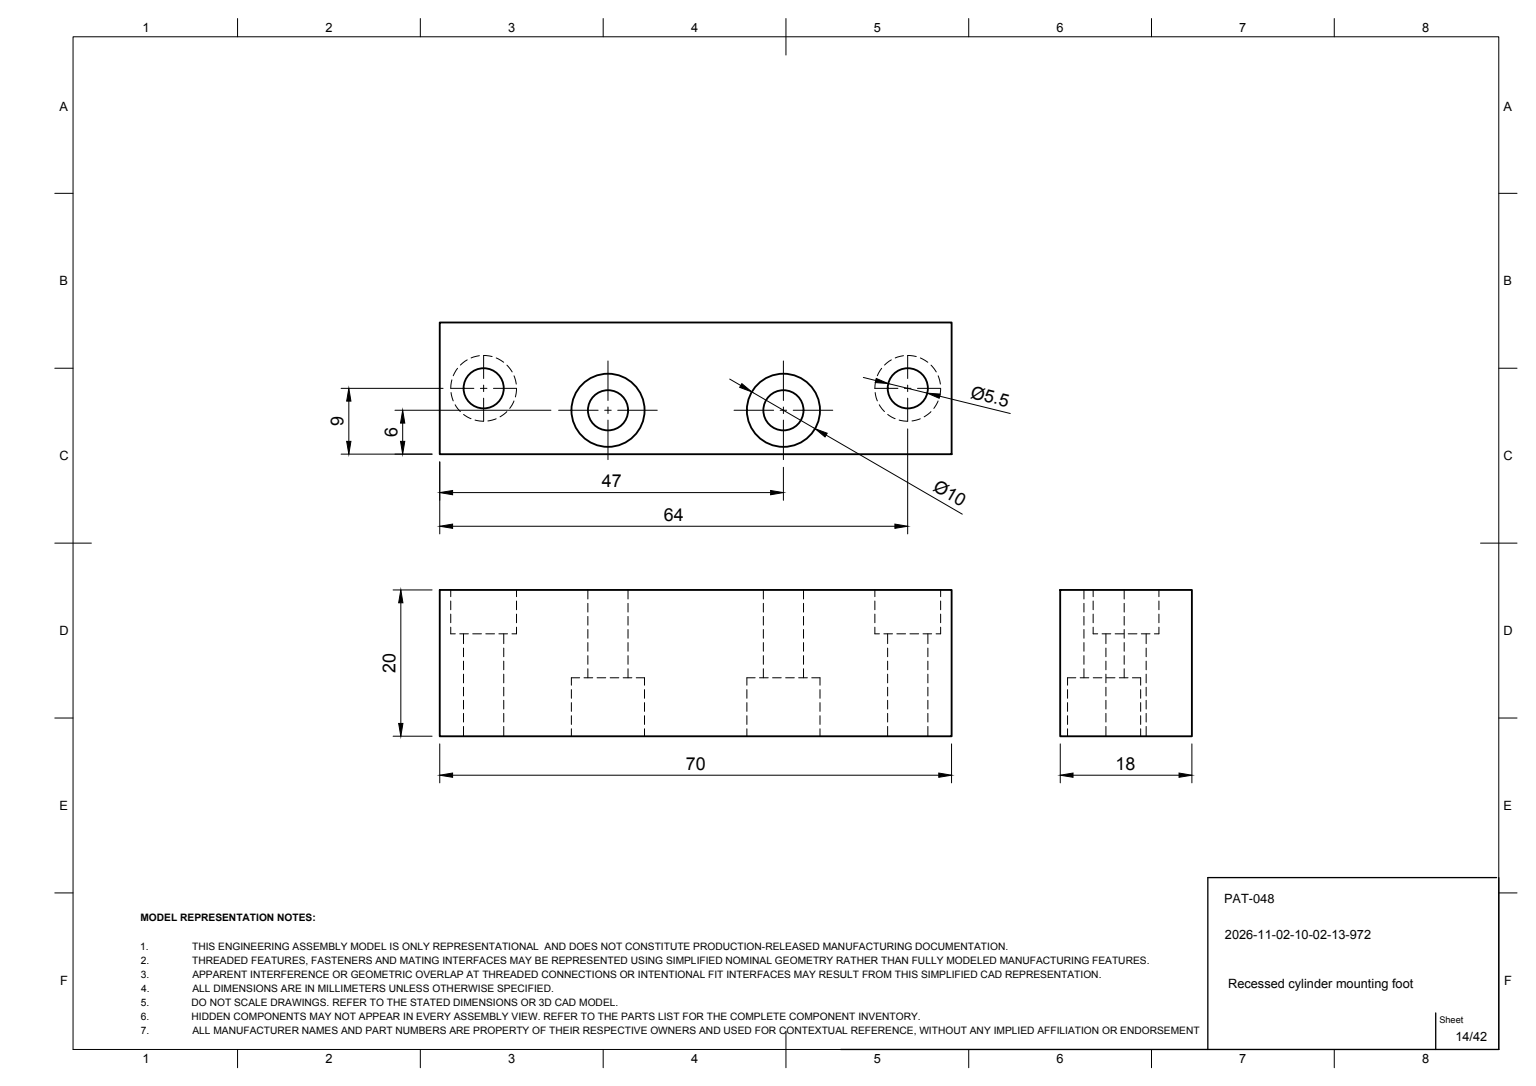
ISO-10303-21;
HEADER;
/* Generated by software containing ST-Developer
 * from STEP Tools, Inc. (www.steptools.com) 
 */

FILE_DESCRIPTION(
/* description */ ('Guided pneumatic stop gate'),
/* implementation_level */ '2;1');

FILE_NAME(
/* name */ 'Recessed cylinder mounting foot.step',
/* time_stamp */ '2026-10-27T21:43:45-07:00',
/* author */ (''),
/* organization */ (''),
/* preprocessor_version */ 'ST-DEVELOPER v20.2',
/* originating_system */ 'Autodesk Translation Framework v15.17.0.0',
/* authorisation */ '');

FILE_SCHEMA (('AUTOMOTIVE_DESIGN { 1 0 10303 214 3 1 1 }'));
ENDSEC;

DATA;
#10=MECHANICAL_DESIGN_GEOMETRIC_PRESENTATION_REPRESENTATION('',(#544),#14392);
#460=SHAPE_REPRESENTATION_RELATIONSHIP('SRR','None',#14594,#502);
#502=ADVANCED_BREP_SHAPE_REPRESENTATION('',(#586),#14356);
#544=STYLED_ITEM('',(#14877),#586);
#586=MANIFOLD_SOLID_BREP('Body1',#7884);
#669=FACE_BOUND('',#1794,.T.);
#670=FACE_BOUND('',#1797,.T.);
#671=FACE_BOUND('',#1802,.T.);
#672=FACE_BOUND('',#1805,.T.);
#673=FACE_BOUND('',#1813,.T.);
#674=FACE_BOUND('',#1814,.T.);
#675=FACE_BOUND('',#1815,.T.);
#676=FACE_BOUND('',#1816,.T.);
#677=FACE_BOUND('',#1818,.T.);
#678=FACE_BOUND('',#1819,.T.);
#679=FACE_BOUND('',#1820,.T.);
#680=FACE_BOUND('',#1821,.T.);
#927=PLANE('',#8666);
#928=PLANE('',#8671);
#929=PLANE('',#8680);
#930=PLANE('',#8685);
#931=PLANE('',#8691);
#932=PLANE('',#8692);
#933=PLANE('',#8693);
#934=PLANE('',#8694);
#935=PLANE('',#8695);
#936=PLANE('',#8696);
#1263=FACE_OUTER_BOUND('',#1792,.T.);
#1264=FACE_OUTER_BOUND('',#1793,.T.);
#1265=FACE_OUTER_BOUND('',#1795,.T.);
#1266=FACE_OUTER_BOUND('',#1796,.T.);
#1267=FACE_OUTER_BOUND('',#1798,.T.);
#1268=FACE_OUTER_BOUND('',#1799,.T.);
#1269=FACE_OUTER_BOUND('',#1800,.T.);
#1270=FACE_OUTER_BOUND('',#1801,.T.);
#1271=FACE_OUTER_BOUND('',#1803,.T.);
#1272=FACE_OUTER_BOUND('',#1804,.T.);
#1273=FACE_OUTER_BOUND('',#1806,.T.);
#1274=FACE_OUTER_BOUND('',#1807,.T.);
#1275=FACE_OUTER_BOUND('',#1808,.T.);
#1276=FACE_OUTER_BOUND('',#1809,.T.);
#1277=FACE_OUTER_BOUND('',#1810,.T.);
#1278=FACE_OUTER_BOUND('',#1811,.T.);
#1279=FACE_OUTER_BOUND('',#1812,.T.);
#1280=FACE_OUTER_BOUND('',#1817,.T.);
#1792=EDGE_LOOP('',(#5898,#5899,#5900,#5901));
#1793=EDGE_LOOP('',(#5902));
#1794=EDGE_LOOP('',(#5903));
#1795=EDGE_LOOP('',(#5904,#5905,#5906,#5907));
#1796=EDGE_LOOP('',(#5908));
#1797=EDGE_LOOP('',(#5909));
#1798=EDGE_LOOP('',(#5910,#5911,#5912,#5913));
#1799=EDGE_LOOP('',(#5914,#5915,#5916,#5917));
#1800=EDGE_LOOP('',(#5918,#5919,#5920,#5921));
#1801=EDGE_LOOP('',(#5922));
#1802=EDGE_LOOP('',(#5923));
#1803=EDGE_LOOP('',(#5924,#5925,#5926,#5927));
#1804=EDGE_LOOP('',(#5928));
#1805=EDGE_LOOP('',(#5929));
#1806=EDGE_LOOP('',(#5930,#5931,#5932,#5933));
#1807=EDGE_LOOP('',(#5934,#5935,#5936,#5937));
#1808=EDGE_LOOP('',(#5938,#5939,#5940,#5941));
#1809=EDGE_LOOP('',(#5942,#5943,#5944,#5945));
#1810=EDGE_LOOP('',(#5946,#5947,#5948,#5949));
#1811=EDGE_LOOP('',(#5950,#5951,#5952,#5953));
#1812=EDGE_LOOP('',(#5954,#5955,#5956,#5957));
#1813=EDGE_LOOP('',(#5958));
#1814=EDGE_LOOP('',(#5959));
#1815=EDGE_LOOP('',(#5960));
#1816=EDGE_LOOP('',(#5961));
#1817=EDGE_LOOP('',(#5962,#5963,#5964,#5965));
#1818=EDGE_LOOP('',(#5966));
#1819=EDGE_LOOP('',(#5967));
#1820=EDGE_LOOP('',(#5968));
#1821=EDGE_LOOP('',(#5969));
#2447=LINE('',#12554,#2992);
#2448=LINE('',#12563,#2993);
#2449=LINE('',#12571,#2994);
#2450=LINE('',#12575,#2995);
#2451=LINE('',#12580,#2996);
#2452=LINE('',#12589,#2997);
#2453=LINE('',#12596,#2998);
#2454=LINE('',#12600,#2999);
#2455=LINE('',#12605,#3000);
#2456=LINE('',#12607,#3001);
#2457=LINE('',#12609,#3002);
#2458=LINE('',#12610,#3003);
#2459=LINE('',#12613,#3004);
#2460=LINE('',#12615,#3005);
#2461=LINE('',#12616,#3006);
#2462=LINE('',#12619,#3007);
#2463=LINE('',#12621,#3008);
#2464=LINE('',#12622,#3009);
#2465=LINE('',#12624,#3010);
#2466=LINE('',#12625,#3011);
#2992=VECTOR('',#10112,0.45);
#2993=VECTOR('',#10123,0.45);
#2994=VECTOR('',#10134,0.275);
#2995=VECTOR('',#10139,0.275);
#2996=VECTOR('',#10144,0.5);
#2997=VECTOR('',#10155,0.5);
#2998=VECTOR('',#10164,0.275);
#2999=VECTOR('',#10169,0.275);
#3000=VECTOR('',#10174,1.);
#3001=VECTOR('',#10175,1.);
#3002=VECTOR('',#10176,1.);
#3003=VECTOR('',#10177,1.);
#3004=VECTOR('',#10180,1.);
#3005=VECTOR('',#10181,1.);
#3006=VECTOR('',#10182,1.);
#3007=VECTOR('',#10185,1.);
#3008=VECTOR('',#10186,1.);
#3009=VECTOR('',#10187,1.);
#3010=VECTOR('',#10190,1.);
#3011=VECTOR('',#10191,1.);
#3476=CIRCLE('',#8664,0.45);
#3477=CIRCLE('',#8665,0.45);
#3478=CIRCLE('',#8667,0.275);
#3479=CIRCLE('',#8669,0.45);
#3480=CIRCLE('',#8670,0.45);
#3481=CIRCLE('',#8672,0.275);
#3482=CIRCLE('',#8674,0.275);
#3483=CIRCLE('',#8676,0.275);
#3484=CIRCLE('',#8678,0.5);
#3485=CIRCLE('',#8679,0.5);
#3486=CIRCLE('',#8681,0.275);
#3487=CIRCLE('',#8683,0.5);
#3488=CIRCLE('',#8684,0.5);
#3489=CIRCLE('',#8686,0.275);
#3490=CIRCLE('',#8688,0.275);
#3491=CIRCLE('',#8690,0.275);
#3919=VERTEX_POINT('',#12551);
#3920=VERTEX_POINT('',#12553);
#3921=VERTEX_POINT('',#12557);
#3922=VERTEX_POINT('',#12560);
#3923=VERTEX_POINT('',#12562);
#3924=VERTEX_POINT('',#12566);
#3925=VERTEX_POINT('',#12569);
#3926=VERTEX_POINT('',#12573);
#3927=VERTEX_POINT('',#12577);
#3928=VERTEX_POINT('',#12579);
#3929=VERTEX_POINT('',#12583);
#3930=VERTEX_POINT('',#12586);
#3931=VERTEX_POINT('',#12588);
#3932=VERTEX_POINT('',#12592);
#3933=VERTEX_POINT('',#12595);
#3934=VERTEX_POINT('',#12599);
#3935=VERTEX_POINT('',#12603);
#3936=VERTEX_POINT('',#12604);
#3937=VERTEX_POINT('',#12606);
#3938=VERTEX_POINT('',#12608);
#3939=VERTEX_POINT('',#12612);
#3940=VERTEX_POINT('',#12614);
#3941=VERTEX_POINT('',#12618);
#3942=VERTEX_POINT('',#12620);
#4647=EDGE_CURVE('',#3919,#3919,#3476,.T.);
#4648=EDGE_CURVE('',#3919,#3920,#2447,.T.);
#4649=EDGE_CURVE('',#3920,#3920,#3477,.T.);
#4650=EDGE_CURVE('',#3921,#3921,#3478,.T.);
#4651=EDGE_CURVE('',#3922,#3922,#3479,.T.);
#4652=EDGE_CURVE('',#3922,#3923,#2448,.T.);
#4653=EDGE_CURVE('',#3923,#3923,#3480,.T.);
#4654=EDGE_CURVE('',#3924,#3924,#3481,.T.);
#4655=EDGE_CURVE('',#3925,#3925,#3482,.T.);
#4656=EDGE_CURVE('',#3925,#3921,#2449,.T.);
#4657=EDGE_CURVE('',#3926,#3926,#3483,.T.);
#4658=EDGE_CURVE('',#3926,#3924,#2450,.T.);
#4659=EDGE_CURVE('',#3927,#3927,#3484,.T.);
#4660=EDGE_CURVE('',#3927,#3928,#2451,.T.);
#4661=EDGE_CURVE('',#3928,#3928,#3485,.T.);
#4662=EDGE_CURVE('',#3929,#3929,#3486,.T.);
#4663=EDGE_CURVE('',#3930,#3930,#3487,.T.);
#4664=EDGE_CURVE('',#3930,#3931,#2452,.T.);
#4665=EDGE_CURVE('',#3931,#3931,#3488,.T.);
#4666=EDGE_CURVE('',#3932,#3932,#3489,.T.);
#4667=EDGE_CURVE('',#3929,#3933,#2453,.T.);
#4668=EDGE_CURVE('',#3933,#3933,#3490,.T.);
#4669=EDGE_CURVE('',#3932,#3934,#2454,.T.);
#4670=EDGE_CURVE('',#3934,#3934,#3491,.T.);
#4671=EDGE_CURVE('',#3935,#3936,#2455,.T.);
#4672=EDGE_CURVE('',#3936,#3937,#2456,.T.);
#4673=EDGE_CURVE('',#3938,#3937,#2457,.T.);
#4674=EDGE_CURVE('',#3935,#3938,#2458,.T.);
#4675=EDGE_CURVE('',#3939,#3935,#2459,.T.);
#4676=EDGE_CURVE('',#3940,#3938,#2460,.T.);
#4677=EDGE_CURVE('',#3939,#3940,#2461,.T.);
#4678=EDGE_CURVE('',#3941,#3939,#2462,.T.);
#4679=EDGE_CURVE('',#3942,#3940,#2463,.T.);
#4680=EDGE_CURVE('',#3941,#3942,#2464,.T.);
#4681=EDGE_CURVE('',#3936,#3941,#2465,.T.);
#4682=EDGE_CURVE('',#3937,#3942,#2466,.T.);
#5898=ORIENTED_EDGE('',*,*,#4647,.F.);
#5899=ORIENTED_EDGE('',*,*,#4648,.T.);
#5900=ORIENTED_EDGE('',*,*,#4649,.F.);
#5901=ORIENTED_EDGE('',*,*,#4648,.F.);
#5902=ORIENTED_EDGE('',*,*,#4647,.T.);
#5903=ORIENTED_EDGE('',*,*,#4650,.F.);
#5904=ORIENTED_EDGE('',*,*,#4651,.F.);
#5905=ORIENTED_EDGE('',*,*,#4652,.T.);
#5906=ORIENTED_EDGE('',*,*,#4653,.F.);
#5907=ORIENTED_EDGE('',*,*,#4652,.F.);
#5908=ORIENTED_EDGE('',*,*,#4651,.T.);
#5909=ORIENTED_EDGE('',*,*,#4654,.F.);
#5910=ORIENTED_EDGE('',*,*,#4655,.F.);
#5911=ORIENTED_EDGE('',*,*,#4656,.T.);
#5912=ORIENTED_EDGE('',*,*,#4650,.T.);
#5913=ORIENTED_EDGE('',*,*,#4656,.F.);
#5914=ORIENTED_EDGE('',*,*,#4657,.F.);
#5915=ORIENTED_EDGE('',*,*,#4658,.T.);
#5916=ORIENTED_EDGE('',*,*,#4654,.T.);
#5917=ORIENTED_EDGE('',*,*,#4658,.F.);
#5918=ORIENTED_EDGE('',*,*,#4659,.F.);
#5919=ORIENTED_EDGE('',*,*,#4660,.T.);
#5920=ORIENTED_EDGE('',*,*,#4661,.T.);
#5921=ORIENTED_EDGE('',*,*,#4660,.F.);
#5922=ORIENTED_EDGE('',*,*,#4661,.F.);
#5923=ORIENTED_EDGE('',*,*,#4662,.F.);
#5924=ORIENTED_EDGE('',*,*,#4663,.F.);
#5925=ORIENTED_EDGE('',*,*,#4664,.T.);
#5926=ORIENTED_EDGE('',*,*,#4665,.T.);
#5927=ORIENTED_EDGE('',*,*,#4664,.F.);
#5928=ORIENTED_EDGE('',*,*,#4665,.F.);
#5929=ORIENTED_EDGE('',*,*,#4666,.F.);
#5930=ORIENTED_EDGE('',*,*,#4662,.T.);
#5931=ORIENTED_EDGE('',*,*,#4667,.T.);
#5932=ORIENTED_EDGE('',*,*,#4668,.F.);
#5933=ORIENTED_EDGE('',*,*,#4667,.F.);
#5934=ORIENTED_EDGE('',*,*,#4666,.T.);
#5935=ORIENTED_EDGE('',*,*,#4669,.T.);
#5936=ORIENTED_EDGE('',*,*,#4670,.F.);
#5937=ORIENTED_EDGE('',*,*,#4669,.F.);
#5938=ORIENTED_EDGE('',*,*,#4671,.T.);
#5939=ORIENTED_EDGE('',*,*,#4672,.T.);
#5940=ORIENTED_EDGE('',*,*,#4673,.F.);
#5941=ORIENTED_EDGE('',*,*,#4674,.F.);
#5942=ORIENTED_EDGE('',*,*,#4675,.T.);
#5943=ORIENTED_EDGE('',*,*,#4674,.T.);
#5944=ORIENTED_EDGE('',*,*,#4676,.F.);
#5945=ORIENTED_EDGE('',*,*,#4677,.F.);
#5946=ORIENTED_EDGE('',*,*,#4678,.T.);
#5947=ORIENTED_EDGE('',*,*,#4677,.T.);
#5948=ORIENTED_EDGE('',*,*,#4679,.F.);
#5949=ORIENTED_EDGE('',*,*,#4680,.F.);
#5950=ORIENTED_EDGE('',*,*,#4681,.T.);
#5951=ORIENTED_EDGE('',*,*,#4680,.T.);
#5952=ORIENTED_EDGE('',*,*,#4682,.F.);
#5953=ORIENTED_EDGE('',*,*,#4672,.F.);
#5954=ORIENTED_EDGE('',*,*,#4682,.T.);
#5955=ORIENTED_EDGE('',*,*,#4679,.T.);
#5956=ORIENTED_EDGE('',*,*,#4676,.T.);
#5957=ORIENTED_EDGE('',*,*,#4673,.T.);
#5958=ORIENTED_EDGE('',*,*,#4649,.T.);
#5959=ORIENTED_EDGE('',*,*,#4653,.T.);
#5960=ORIENTED_EDGE('',*,*,#4668,.T.);
#5961=ORIENTED_EDGE('',*,*,#4670,.T.);
#5962=ORIENTED_EDGE('',*,*,#4681,.F.);
#5963=ORIENTED_EDGE('',*,*,#4671,.F.);
#5964=ORIENTED_EDGE('',*,*,#4675,.F.);
#5965=ORIENTED_EDGE('',*,*,#4678,.F.);
#5966=ORIENTED_EDGE('',*,*,#4655,.T.);
#5967=ORIENTED_EDGE('',*,*,#4657,.T.);
#5968=ORIENTED_EDGE('',*,*,#4659,.T.);
#5969=ORIENTED_EDGE('',*,*,#4663,.T.);
#7289=CYLINDRICAL_SURFACE('',#8663,0.45);
#7290=CYLINDRICAL_SURFACE('',#8668,0.45);
#7291=CYLINDRICAL_SURFACE('',#8673,0.275);
#7292=CYLINDRICAL_SURFACE('',#8675,0.275);
#7293=CYLINDRICAL_SURFACE('',#8677,0.5);
#7294=CYLINDRICAL_SURFACE('',#8682,0.5);
#7295=CYLINDRICAL_SURFACE('',#8687,0.275);
#7296=CYLINDRICAL_SURFACE('',#8689,0.275);
#7545=ADVANCED_FACE('',(#1263),#7289,.F.);
#7546=ADVANCED_FACE('',(#1264,#669),#927,.T.);
#7547=ADVANCED_FACE('',(#1265),#7290,.F.);
#7548=ADVANCED_FACE('',(#1266,#670),#928,.T.);
#7549=ADVANCED_FACE('',(#1267),#7291,.F.);
#7550=ADVANCED_FACE('',(#1268),#7292,.F.);
#7551=ADVANCED_FACE('',(#1269),#7293,.F.);
#7552=ADVANCED_FACE('',(#1270,#671),#929,.F.);
#7553=ADVANCED_FACE('',(#1271),#7294,.F.);
#7554=ADVANCED_FACE('',(#1272,#672),#930,.F.);
#7555=ADVANCED_FACE('',(#1273),#7295,.F.);
#7556=ADVANCED_FACE('',(#1274),#7296,.F.);
#7557=ADVANCED_FACE('',(#1275),#931,.T.);
#7558=ADVANCED_FACE('',(#1276),#932,.T.);
#7559=ADVANCED_FACE('',(#1277),#933,.T.);
#7560=ADVANCED_FACE('',(#1278),#934,.T.);
#7561=ADVANCED_FACE('',(#1279,#673,#674,#675,#676),#935,.T.);
#7562=ADVANCED_FACE('',(#1280,#677,#678,#679,#680),#936,.F.);
#7884=CLOSED_SHELL('',(#7545,#7546,#7547,#7548,#7549,#7550,#7551,#7552,
#7553,#7554,#7555,#7556,#7557,#7558,#7559,#7560,#7561,#7562));
#8662=AXIS2_PLACEMENT_3D('',#12549,#10106,#10107);
#8663=AXIS2_PLACEMENT_3D('',#12550,#10108,#10109);
#8664=AXIS2_PLACEMENT_3D('',#12552,#10110,#10111);
#8665=AXIS2_PLACEMENT_3D('',#12555,#10113,#10114);
#8666=AXIS2_PLACEMENT_3D('',#12556,#10115,#10116);
#8667=AXIS2_PLACEMENT_3D('',#12558,#10117,#10118);
#8668=AXIS2_PLACEMENT_3D('',#12559,#10119,#10120);
#8669=AXIS2_PLACEMENT_3D('',#12561,#10121,#10122);
#8670=AXIS2_PLACEMENT_3D('',#12564,#10124,#10125);
#8671=AXIS2_PLACEMENT_3D('',#12565,#10126,#10127);
#8672=AXIS2_PLACEMENT_3D('',#12567,#10128,#10129);
#8673=AXIS2_PLACEMENT_3D('',#12568,#10130,#10131);
#8674=AXIS2_PLACEMENT_3D('',#12570,#10132,#10133);
#8675=AXIS2_PLACEMENT_3D('',#12572,#10135,#10136);
#8676=AXIS2_PLACEMENT_3D('',#12574,#10137,#10138);
#8677=AXIS2_PLACEMENT_3D('',#12576,#10140,#10141);
#8678=AXIS2_PLACEMENT_3D('',#12578,#10142,#10143);
#8679=AXIS2_PLACEMENT_3D('',#12581,#10145,#10146);
#8680=AXIS2_PLACEMENT_3D('',#12582,#10147,#10148);
#8681=AXIS2_PLACEMENT_3D('',#12584,#10149,#10150);
#8682=AXIS2_PLACEMENT_3D('',#12585,#10151,#10152);
#8683=AXIS2_PLACEMENT_3D('',#12587,#10153,#10154);
#8684=AXIS2_PLACEMENT_3D('',#12590,#10156,#10157);
#8685=AXIS2_PLACEMENT_3D('',#12591,#10158,#10159);
#8686=AXIS2_PLACEMENT_3D('',#12593,#10160,#10161);
#8687=AXIS2_PLACEMENT_3D('',#12594,#10162,#10163);
#8688=AXIS2_PLACEMENT_3D('',#12597,#10165,#10166);
#8689=AXIS2_PLACEMENT_3D('',#12598,#10167,#10168);
#8690=AXIS2_PLACEMENT_3D('',#12601,#10170,#10171);
#8691=AXIS2_PLACEMENT_3D('',#12602,#10172,#10173);
#8692=AXIS2_PLACEMENT_3D('',#12611,#10178,#10179);
#8693=AXIS2_PLACEMENT_3D('',#12617,#10183,#10184);
#8694=AXIS2_PLACEMENT_3D('',#12623,#10188,#10189);
#8695=AXIS2_PLACEMENT_3D('',#12626,#10192,#10193);
#8696=AXIS2_PLACEMENT_3D('',#12627,#10194,#10195);
#10106=DIRECTION('axis',(0.,0.,1.));
#10107=DIRECTION('refdir',(1.,0.,0.));
#10108=DIRECTION('center_axis',(0.,0.,1.));
#10109=DIRECTION('ref_axis',(1.,0.,0.));
#10110=DIRECTION('center_axis',(0.,0.,1.));
#10111=DIRECTION('ref_axis',(1.,0.,0.));
#10112=DIRECTION('',(0.,0.,1.));
#10113=DIRECTION('center_axis',(0.,0.,-1.));
#10114=DIRECTION('ref_axis',(1.,0.,0.));
#10115=DIRECTION('center_axis',(0.,0.,1.));
#10116=DIRECTION('ref_axis',(1.,0.,0.));
#10117=DIRECTION('center_axis',(0.,0.,1.));
#10118=DIRECTION('ref_axis',(1.,0.,0.));
#10119=DIRECTION('center_axis',(0.,0.,1.));
#10120=DIRECTION('ref_axis',(1.,0.,0.));
#10121=DIRECTION('center_axis',(0.,0.,1.));
#10122=DIRECTION('ref_axis',(1.,0.,0.));
#10123=DIRECTION('',(0.,0.,1.));
#10124=DIRECTION('center_axis',(0.,0.,-1.));
#10125=DIRECTION('ref_axis',(1.,0.,0.));
#10126=DIRECTION('center_axis',(0.,0.,1.));
#10127=DIRECTION('ref_axis',(1.,0.,0.));
#10128=DIRECTION('center_axis',(0.,0.,1.));
#10129=DIRECTION('ref_axis',(1.,0.,0.));
#10130=DIRECTION('center_axis',(0.,0.,1.));
#10131=DIRECTION('ref_axis',(1.,0.,0.));
#10132=DIRECTION('center_axis',(0.,0.,1.));
#10133=DIRECTION('ref_axis',(1.,0.,0.));
#10134=DIRECTION('',(0.,0.,1.));
#10135=DIRECTION('center_axis',(0.,0.,1.));
#10136=DIRECTION('ref_axis',(1.,0.,0.));
#10137=DIRECTION('center_axis',(0.,0.,1.));
#10138=DIRECTION('ref_axis',(1.,0.,0.));
#10139=DIRECTION('',(0.,0.,1.));
#10140=DIRECTION('center_axis',(0.,0.,1.));
#10141=DIRECTION('ref_axis',(1.,0.,0.));
#10142=DIRECTION('center_axis',(0.,0.,1.));
#10143=DIRECTION('ref_axis',(1.,0.,0.));
#10144=DIRECTION('',(0.,0.,1.));
#10145=DIRECTION('center_axis',(0.,0.,1.));
#10146=DIRECTION('ref_axis',(1.,0.,0.));
#10147=DIRECTION('center_axis',(0.,0.,1.));
#10148=DIRECTION('ref_axis',(1.,0.,0.));
#10149=DIRECTION('center_axis',(0.,0.,-1.));
#10150=DIRECTION('ref_axis',(1.,0.,0.));
#10151=DIRECTION('center_axis',(0.,0.,1.));
#10152=DIRECTION('ref_axis',(1.,0.,0.));
#10153=DIRECTION('center_axis',(0.,0.,1.));
#10154=DIRECTION('ref_axis',(1.,0.,0.));
#10155=DIRECTION('',(0.,0.,1.));
#10156=DIRECTION('center_axis',(0.,0.,1.));
#10157=DIRECTION('ref_axis',(1.,0.,0.));
#10158=DIRECTION('center_axis',(0.,0.,1.));
#10159=DIRECTION('ref_axis',(1.,0.,0.));
#10160=DIRECTION('center_axis',(0.,0.,-1.));
#10161=DIRECTION('ref_axis',(1.,0.,0.));
#10162=DIRECTION('center_axis',(0.,0.,1.));
#10163=DIRECTION('ref_axis',(1.,0.,0.));
#10164=DIRECTION('',(0.,0.,1.));
#10165=DIRECTION('center_axis',(0.,0.,-1.));
#10166=DIRECTION('ref_axis',(1.,0.,0.));
#10167=DIRECTION('center_axis',(0.,0.,1.));
#10168=DIRECTION('ref_axis',(1.,0.,0.));
#10169=DIRECTION('',(0.,0.,1.));
#10170=DIRECTION('center_axis',(0.,0.,-1.));
#10171=DIRECTION('ref_axis',(1.,0.,0.));
#10172=DIRECTION('center_axis',(0.,1.,0.));
#10173=DIRECTION('ref_axis',(-1.,0.,0.));
#10174=DIRECTION('',(-1.,0.,0.));
#10175=DIRECTION('',(0.,0.,1.));
#10176=DIRECTION('',(-1.,0.,0.));
#10177=DIRECTION('',(0.,0.,1.));
#10178=DIRECTION('center_axis',(1.,0.,0.));
#10179=DIRECTION('ref_axis',(0.,1.,0.));
#10180=DIRECTION('',(0.,1.,0.));
#10181=DIRECTION('',(0.,1.,0.));
#10182=DIRECTION('',(0.,0.,1.));
#10183=DIRECTION('center_axis',(0.,-1.,0.));
#10184=DIRECTION('ref_axis',(1.,0.,0.));
#10185=DIRECTION('',(1.,0.,0.));
#10186=DIRECTION('',(1.,0.,0.));
#10187=DIRECTION('',(0.,0.,1.));
#10188=DIRECTION('center_axis',(-1.,0.,0.));
#10189=DIRECTION('ref_axis',(0.,-1.,0.));
#10190=DIRECTION('',(0.,-1.,0.));
#10191=DIRECTION('',(0.,-1.,0.));
#10192=DIRECTION('center_axis',(0.,0.,1.));
#10193=DIRECTION('ref_axis',(1.,0.,0.));
#10194=DIRECTION('center_axis',(0.,0.,1.));
#10195=DIRECTION('ref_axis',(1.,0.,0.));
#12549=CARTESIAN_POINT('',(0.,0.,0.));
#12550=CARTESIAN_POINT('Origin',(-2.9,0.9,1.4));
#12551=CARTESIAN_POINT('',(-3.35,0.9,1.4));
#12552=CARTESIAN_POINT('Origin',(-2.9,0.9,1.4));
#12553=CARTESIAN_POINT('',(-3.35,0.9,2.));
#12554=CARTESIAN_POINT('',(-3.35,0.9,1.4));
#12555=CARTESIAN_POINT('Origin',(-2.9,0.9,2.));
#12556=CARTESIAN_POINT('Origin',(-2.9,0.9,1.4));
#12557=CARTESIAN_POINT('',(-3.175,0.9,1.4));
#12558=CARTESIAN_POINT('Origin',(-2.9,0.9,1.4));
#12559=CARTESIAN_POINT('Origin',(2.9,0.9,1.4));
#12560=CARTESIAN_POINT('',(2.45,0.9,1.4));
#12561=CARTESIAN_POINT('Origin',(2.9,0.9,1.4));
#12562=CARTESIAN_POINT('',(2.45,0.9,2.));
#12563=CARTESIAN_POINT('',(2.45,0.9,1.4));
#12564=CARTESIAN_POINT('Origin',(2.9,0.9,2.));
#12565=CARTESIAN_POINT('Origin',(2.9,0.9,1.4));
#12566=CARTESIAN_POINT('',(2.625,0.9,1.4));
#12567=CARTESIAN_POINT('Origin',(2.9,0.9,1.4));
#12568=CARTESIAN_POINT('Origin',(-2.9,0.9,-0.1));
#12569=CARTESIAN_POINT('',(-3.175,0.9,0.));
#12570=CARTESIAN_POINT('Origin',(-2.9,0.9,0.));
#12571=CARTESIAN_POINT('',(-3.175,0.9,-0.1));
#12572=CARTESIAN_POINT('Origin',(2.9,0.9,-0.1));
#12573=CARTESIAN_POINT('',(2.625,0.9,0.));
#12574=CARTESIAN_POINT('Origin',(2.9,0.9,0.));
#12575=CARTESIAN_POINT('',(2.625,0.9,-0.1));
#12576=CARTESIAN_POINT('Origin',(-1.2,0.6,-0.1));
#12577=CARTESIAN_POINT('',(-1.7,0.6,0.));
#12578=CARTESIAN_POINT('Origin',(-1.2,0.6,0.));
#12579=CARTESIAN_POINT('',(-1.7,0.6,0.8));
#12580=CARTESIAN_POINT('',(-1.7,0.6,-0.1));
#12581=CARTESIAN_POINT('Origin',(-1.2,0.6,0.8));
#12582=CARTESIAN_POINT('Origin',(-1.2,0.6,0.8));
#12583=CARTESIAN_POINT('',(-1.475,0.6,0.8));
#12584=CARTESIAN_POINT('Origin',(-1.2,0.6,0.8));
#12585=CARTESIAN_POINT('Origin',(1.2,0.6,-0.1));
#12586=CARTESIAN_POINT('',(0.7,0.6,0.));
#12587=CARTESIAN_POINT('Origin',(1.2,0.6,0.));
#12588=CARTESIAN_POINT('',(0.7,0.6,0.8));
#12589=CARTESIAN_POINT('',(0.7,0.6,-0.1));
#12590=CARTESIAN_POINT('Origin',(1.2,0.6,0.8));
#12591=CARTESIAN_POINT('Origin',(1.2,0.6,0.8));
#12592=CARTESIAN_POINT('',(0.925,0.6,0.8));
#12593=CARTESIAN_POINT('Origin',(1.2,0.6,0.8));
#12594=CARTESIAN_POINT('Origin',(-1.2,0.6,-0.1));
#12595=CARTESIAN_POINT('',(-1.475,0.6,2.));
#12596=CARTESIAN_POINT('',(-1.475,0.6,-0.1));
#12597=CARTESIAN_POINT('Origin',(-1.2,0.6,2.));
#12598=CARTESIAN_POINT('Origin',(1.2,0.6,-0.1));
#12599=CARTESIAN_POINT('',(0.925,0.6,2.));
#12600=CARTESIAN_POINT('',(0.925,0.6,-0.1));
#12601=CARTESIAN_POINT('Origin',(1.2,0.6,2.));
#12602=CARTESIAN_POINT('Origin',(3.5,1.8,0.));
#12603=CARTESIAN_POINT('',(3.5,1.8,0.));
#12604=CARTESIAN_POINT('',(-3.5,1.8,0.));
#12605=CARTESIAN_POINT('',(3.5,1.8,0.));
#12606=CARTESIAN_POINT('',(-3.5,1.8,2.));
#12607=CARTESIAN_POINT('',(-3.5,1.8,0.));
#12608=CARTESIAN_POINT('',(3.5,1.8,2.));
#12609=CARTESIAN_POINT('',(3.5,1.8,2.));
#12610=CARTESIAN_POINT('',(3.5,1.8,0.));
#12611=CARTESIAN_POINT('Origin',(3.5,0.,0.));
#12612=CARTESIAN_POINT('',(3.5,0.,0.));
#12613=CARTESIAN_POINT('',(3.5,0.,0.));
#12614=CARTESIAN_POINT('',(3.5,0.,2.));
#12615=CARTESIAN_POINT('',(3.5,0.,2.));
#12616=CARTESIAN_POINT('',(3.5,0.,0.));
#12617=CARTESIAN_POINT('Origin',(-3.5,0.,0.));
#12618=CARTESIAN_POINT('',(-3.5,0.,0.));
#12619=CARTESIAN_POINT('',(-3.5,0.,0.));
#12620=CARTESIAN_POINT('',(-3.5,0.,2.));
#12621=CARTESIAN_POINT('',(-3.5,0.,2.));
#12622=CARTESIAN_POINT('',(-3.5,0.,0.));
#12623=CARTESIAN_POINT('Origin',(-3.5,1.8,0.));
#12624=CARTESIAN_POINT('',(-3.5,1.8,0.));
#12625=CARTESIAN_POINT('',(-3.5,1.8,2.));
#12626=CARTESIAN_POINT('Origin',(0.,0.9,2.));
#12627=CARTESIAN_POINT('Origin',(0.,0.9,0.));
#14308=UNCERTAINTY_MEASURE_WITH_UNIT(LENGTH_MEASURE(0.001),#14393,
'DISTANCE_ACCURACY_VALUE',
'Maximum model space distance between geometric entities at asserted c
onnectivities');
#14344=UNCERTAINTY_MEASURE_WITH_UNIT(LENGTH_MEASURE(0.001),#14393,
'DISTANCE_ACCURACY_VALUE',
'Maximum model space distance between geometric entities at asserted c
onnectivities');
#14356=(
GEOMETRIC_REPRESENTATION_CONTEXT(3)
GLOBAL_UNCERTAINTY_ASSIGNED_CONTEXT((#14308))
GLOBAL_UNIT_ASSIGNED_CONTEXT((#14393,#14395,#14396))
REPRESENTATION_CONTEXT('','3D')
);
#14392=(
GEOMETRIC_REPRESENTATION_CONTEXT(3)
GLOBAL_UNCERTAINTY_ASSIGNED_CONTEXT((#14344))
GLOBAL_UNIT_ASSIGNED_CONTEXT((#14393,#14395,#14396))
REPRESENTATION_CONTEXT('','3D')
);
#14393=(
LENGTH_UNIT()
NAMED_UNIT(*)
SI_UNIT(.CENTI.,.METRE.)
);
#14395=(
NAMED_UNIT(*)
PLANE_ANGLE_UNIT()
SI_UNIT($,.RADIAN.)
);
#14396=(
NAMED_UNIT(*)
SI_UNIT($,.STERADIAN.)
SOLID_ANGLE_UNIT()
);
#14408=SHAPE_DEFINITION_REPRESENTATION(#14455,#14594);
#14455=PRODUCT_DEFINITION_SHAPE('',$,#14642);
#14594=SHAPE_REPRESENTATION('',(#8662),#14356);
#14630=PRODUCT_DEFINITION_CONTEXT('part definition',#14773,'design');
#14642=PRODUCT_DEFINITION('Recessed cylinder mounting foot',
'Recessed cylinder mounting foot',#14689,#14630);
#14689=PRODUCT_DEFINITION_FORMATION('',$,#14786);
#14773=APPLICATION_CONTEXT(
'Core Data for Automotive Mechanical Design Process');
#14774=PRODUCT_CONTEXT('part definition',#14773,'mechanical');
#14786=PRODUCT('Recessed cylinder mounting foot',
'Recessed cylinder mounting foot','Recessed cylinder mounting foot',(#14774));
#14871=COLOUR_RGB('Light Blue',0.38,0.62,0.78);
#14872=FILL_AREA_STYLE_COLOUR('',#14871);
#14873=FILL_AREA_STYLE('',(#14872));
#14874=SURFACE_STYLE_FILL_AREA(#14873);
#14875=SURFACE_SIDE_STYLE('',(#14874));
#14876=SURFACE_STYLE_USAGE(.BOTH.,#14875);
#14877=PRESENTATION_STYLE_ASSIGNMENT((#14876));
ENDSEC;
END-ISO-10303-21;
